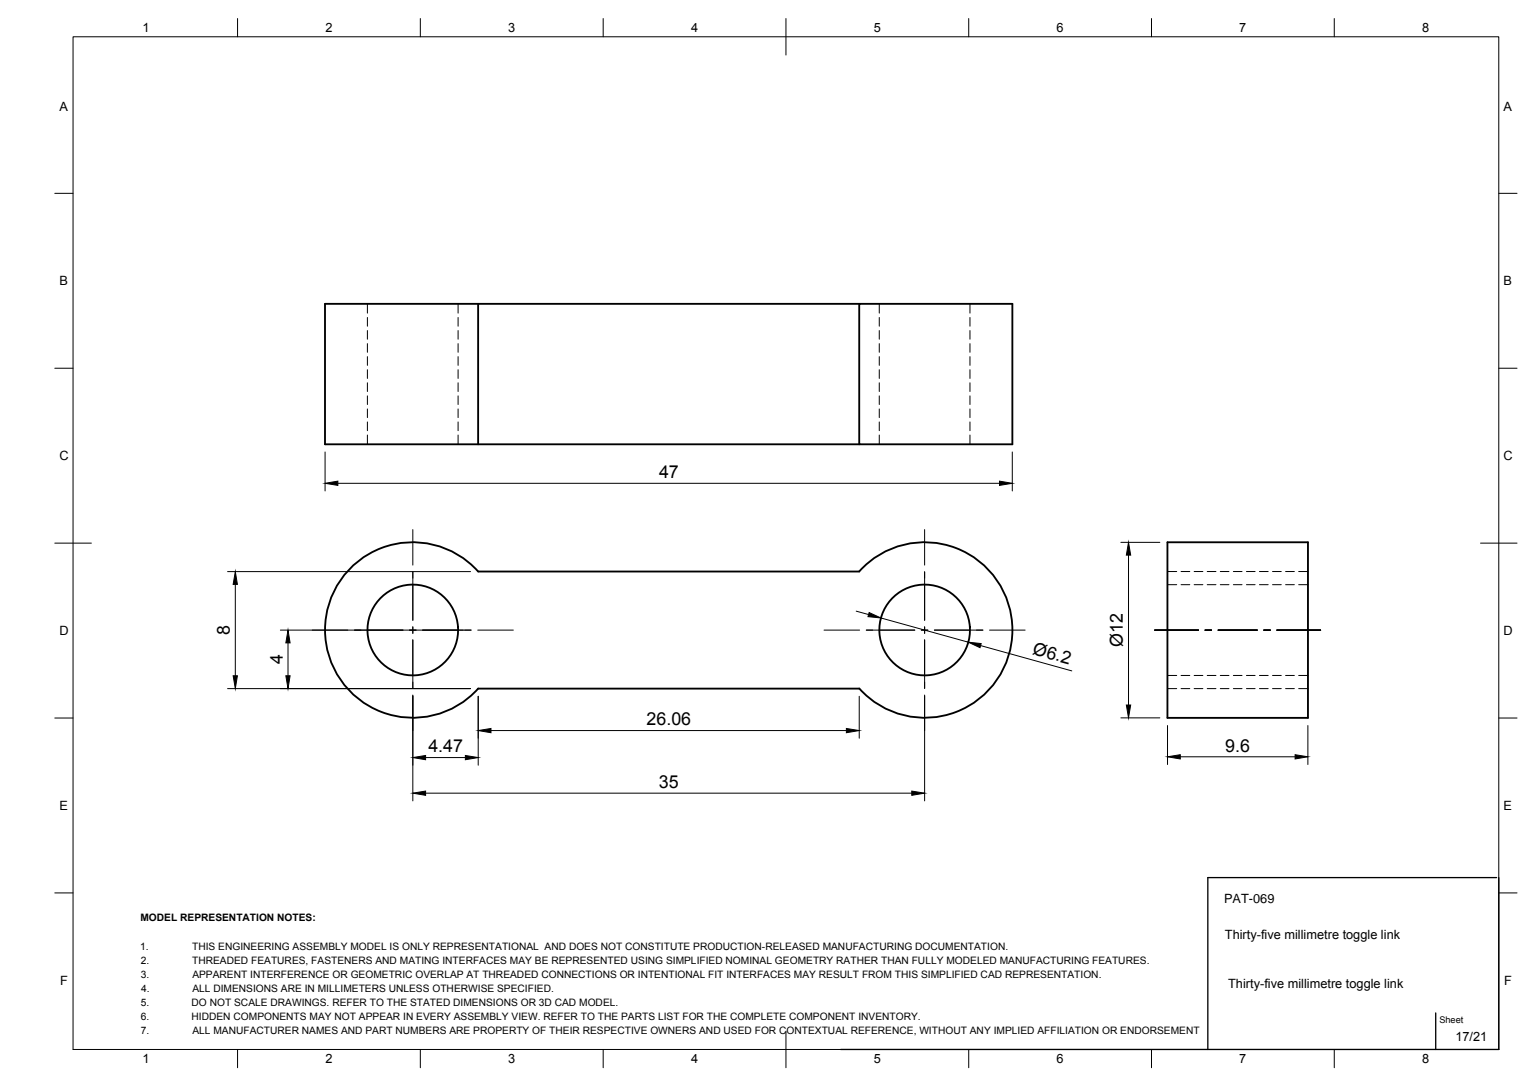
ISO-10303-21;
HEADER;
/* Generated by software containing ST-Developer
 * from STEP Tools, Inc. (www.steptools.com) 
 */

FILE_DESCRIPTION(
/* description */ ('Located fixture plate with toggle clamp'),
/* implementation_level */ '2;1');

FILE_NAME(
/* name */ 'Thirty-five millimetre toggle link.step',
/* time_stamp */ '2026-10-27T21:36:12-07:00',
/* author */ (''),
/* organization */ (''),
/* preprocessor_version */ 'ST-DEVELOPER v20.2',
/* originating_system */ 'Autodesk Translation Framework v15.17.0.0',
/* authorisation */ '');

FILE_SCHEMA (('AUTOMOTIVE_DESIGN { 1 0 10303 214 3 1 1 }'));
ENDSEC;

DATA;
#10=MECHANICAL_DESIGN_GEOMETRIC_PRESENTATION_REPRESENTATION('',(#336),#9285);
#288=SHAPE_REPRESENTATION_RELATIONSHIP('SRR','None',#9413,#312);
#312=ADVANCED_BREP_SHAPE_REPRESENTATION('',(#357),#9275);
#336=STYLED_ITEM('',(#9626),#357);
#357=MANIFOLD_SOLID_BREP('Body1',#5187);
#466=FACE_BOUND('',#1297,.T.);
#467=FACE_BOUND('',#1298,.T.);
#468=FACE_BOUND('',#1302,.T.);
#469=FACE_BOUND('',#1303,.T.);
#628=PLANE('',#5867);
#629=PLANE('',#5868);
#630=PLANE('',#5870);
#631=PLANE('',#5873);
#897=FACE_OUTER_BOUND('',#1292,.T.);
#898=FACE_OUTER_BOUND('',#1293,.T.);
#899=FACE_OUTER_BOUND('',#1294,.T.);
#900=FACE_OUTER_BOUND('',#1295,.T.);
#901=FACE_OUTER_BOUND('',#1296,.T.);
#902=FACE_OUTER_BOUND('',#1299,.T.);
#903=FACE_OUTER_BOUND('',#1300,.T.);
#904=FACE_OUTER_BOUND('',#1301,.T.);
#1292=EDGE_LOOP('',(#4498,#4499,#4500,#4501));
#1293=EDGE_LOOP('',(#4502,#4503,#4504,#4505));
#1294=EDGE_LOOP('',(#4506,#4507,#4508,#4509));
#1295=EDGE_LOOP('',(#4510,#4511,#4512,#4513));
#1296=EDGE_LOOP('',(#4514,#4515,#4516,#4517));
#1297=EDGE_LOOP('',(#4518));
#1298=EDGE_LOOP('',(#4519));
#1299=EDGE_LOOP('',(#4520,#4521,#4522,#4523));
#1300=EDGE_LOOP('',(#4524,#4525,#4526,#4527));
#1301=EDGE_LOOP('',(#4528,#4529,#4530,#4531));
#1302=EDGE_LOOP('',(#4532));
#1303=EDGE_LOOP('',(#4533));
#1536=CIRCLE('',#5859,0.31);
#1537=CIRCLE('',#5860,0.31);
#1538=CIRCLE('',#5862,0.31);
#1539=CIRCLE('',#5863,0.31);
#1540=CIRCLE('',#5865,0.6);
#1541=CIRCLE('',#5866,0.6);
#1542=CIRCLE('',#5869,0.6);
#1543=CIRCLE('',#5872,0.6);
#1913=LINE('',#8707,#2323);
#1914=LINE('',#8713,#2324);
#1915=LINE('',#8718,#2325);
#1916=LINE('',#8722,#2326);
#1917=LINE('',#8726,#2327);
#1918=LINE('',#8728,#2328);
#1919=LINE('',#8729,#2329);
#1920=LINE('',#8732,#2330);
#1921=LINE('',#8736,#2331);
#1922=LINE('',#8737,#2332);
#2323=VECTOR('',#7159,0.31);
#2324=VECTOR('',#7166,0.31);
#2325=VECTOR('',#7171,1.);
#2326=VECTOR('',#7174,1.);
#2327=VECTOR('',#7179,1.);
#2328=VECTOR('',#7180,1.);
#2329=VECTOR('',#7181,1.);
#2330=VECTOR('',#7184,1.);
#2331=VECTOR('',#7189,1.);
#2332=VECTOR('',#7190,1.);
#2734=VERTEX_POINT('',#8704);
#2735=VERTEX_POINT('',#8706);
#2736=VERTEX_POINT('',#8710);
#2737=VERTEX_POINT('',#8712);
#2738=VERTEX_POINT('',#8716);
#2739=VERTEX_POINT('',#8717);
#2740=VERTEX_POINT('',#8719);
#2741=VERTEX_POINT('',#8721);
#2742=VERTEX_POINT('',#8725);
#2743=VERTEX_POINT('',#8727);
#2744=VERTEX_POINT('',#8731);
#2745=VERTEX_POINT('',#8735);
#3337=EDGE_CURVE('',#2734,#2734,#1536,.T.);
#3338=EDGE_CURVE('',#2734,#2735,#1913,.T.);
#3339=EDGE_CURVE('',#2735,#2735,#1537,.T.);
#3340=EDGE_CURVE('',#2736,#2736,#1538,.T.);
#3341=EDGE_CURVE('',#2736,#2737,#1914,.T.);
#3342=EDGE_CURVE('',#2737,#2737,#1539,.T.);
#3343=EDGE_CURVE('',#2738,#2739,#1915,.T.);
#3344=EDGE_CURVE('',#2740,#2738,#1540,.T.);
#3345=EDGE_CURVE('',#2741,#2740,#1916,.T.);
#3346=EDGE_CURVE('',#2741,#2739,#1541,.T.);
#3347=EDGE_CURVE('',#2739,#2742,#1917,.T.);
#3348=EDGE_CURVE('',#2743,#2742,#1918,.T.);
#3349=EDGE_CURVE('',#2738,#2743,#1919,.T.);
#3350=EDGE_CURVE('',#2744,#2741,#1920,.T.);
#3351=EDGE_CURVE('',#2742,#2744,#1542,.T.);
#3352=EDGE_CURVE('',#2745,#2740,#1921,.T.);
#3353=EDGE_CURVE('',#2744,#2745,#1922,.T.);
#3354=EDGE_CURVE('',#2743,#2745,#1543,.T.);
#4498=ORIENTED_EDGE('',*,*,#3337,.F.);
#4499=ORIENTED_EDGE('',*,*,#3338,.T.);
#4500=ORIENTED_EDGE('',*,*,#3339,.F.);
#4501=ORIENTED_EDGE('',*,*,#3338,.F.);
#4502=ORIENTED_EDGE('',*,*,#3340,.F.);
#4503=ORIENTED_EDGE('',*,*,#3341,.T.);
#4504=ORIENTED_EDGE('',*,*,#3342,.F.);
#4505=ORIENTED_EDGE('',*,*,#3341,.F.);
#4506=ORIENTED_EDGE('',*,*,#3343,.F.);
#4507=ORIENTED_EDGE('',*,*,#3344,.F.);
#4508=ORIENTED_EDGE('',*,*,#3345,.F.);
#4509=ORIENTED_EDGE('',*,*,#3346,.T.);
#4510=ORIENTED_EDGE('',*,*,#3343,.T.);
#4511=ORIENTED_EDGE('',*,*,#3347,.T.);
#4512=ORIENTED_EDGE('',*,*,#3348,.F.);
#4513=ORIENTED_EDGE('',*,*,#3349,.F.);
#4514=ORIENTED_EDGE('',*,*,#3346,.F.);
#4515=ORIENTED_EDGE('',*,*,#3350,.F.);
#4516=ORIENTED_EDGE('',*,*,#3351,.F.);
#4517=ORIENTED_EDGE('',*,*,#3347,.F.);
#4518=ORIENTED_EDGE('',*,*,#3337,.T.);
#4519=ORIENTED_EDGE('',*,*,#3340,.T.);
#4520=ORIENTED_EDGE('',*,*,#3345,.T.);
#4521=ORIENTED_EDGE('',*,*,#3352,.F.);
#4522=ORIENTED_EDGE('',*,*,#3353,.F.);
#4523=ORIENTED_EDGE('',*,*,#3350,.T.);
#4524=ORIENTED_EDGE('',*,*,#3348,.T.);
#4525=ORIENTED_EDGE('',*,*,#3351,.T.);
#4526=ORIENTED_EDGE('',*,*,#3353,.T.);
#4527=ORIENTED_EDGE('',*,*,#3354,.F.);
#4528=ORIENTED_EDGE('',*,*,#3349,.T.);
#4529=ORIENTED_EDGE('',*,*,#3354,.T.);
#4530=ORIENTED_EDGE('',*,*,#3352,.T.);
#4531=ORIENTED_EDGE('',*,*,#3344,.T.);
#4532=ORIENTED_EDGE('',*,*,#3339,.T.);
#4533=ORIENTED_EDGE('',*,*,#3342,.T.);
#4855=CYLINDRICAL_SURFACE('',#5858,0.31);
#4856=CYLINDRICAL_SURFACE('',#5861,0.31);
#4857=CYLINDRICAL_SURFACE('',#5864,0.6);
#4858=CYLINDRICAL_SURFACE('',#5871,0.6);
#5098=ADVANCED_FACE('',(#897),#4855,.F.);
#5099=ADVANCED_FACE('',(#898),#4856,.F.);
#5100=ADVANCED_FACE('',(#899),#4857,.T.);
#5101=ADVANCED_FACE('',(#900),#628,.T.);
#5102=ADVANCED_FACE('',(#901,#466,#467),#629,.F.);
#5103=ADVANCED_FACE('',(#902),#630,.T.);
#5104=ADVANCED_FACE('',(#903),#4858,.T.);
#5105=ADVANCED_FACE('',(#904,#468,#469),#631,.T.);
#5187=CLOSED_SHELL('',(#5098,#5099,#5100,#5101,#5102,#5103,#5104,#5105));
#5857=AXIS2_PLACEMENT_3D('',#8702,#7153,#7154);
#5858=AXIS2_PLACEMENT_3D('',#8703,#7155,#7156);
#5859=AXIS2_PLACEMENT_3D('',#8705,#7157,#7158);
#5860=AXIS2_PLACEMENT_3D('',#8708,#7160,#7161);
#5861=AXIS2_PLACEMENT_3D('',#8709,#7162,#7163);
#5862=AXIS2_PLACEMENT_3D('',#8711,#7164,#7165);
#5863=AXIS2_PLACEMENT_3D('',#8714,#7167,#7168);
#5864=AXIS2_PLACEMENT_3D('',#8715,#7169,#7170);
#5865=AXIS2_PLACEMENT_3D('',#8720,#7172,#7173);
#5866=AXIS2_PLACEMENT_3D('',#8723,#7175,#7176);
#5867=AXIS2_PLACEMENT_3D('',#8724,#7177,#7178);
#5868=AXIS2_PLACEMENT_3D('',#8730,#7182,#7183);
#5869=AXIS2_PLACEMENT_3D('',#8733,#7185,#7186);
#5870=AXIS2_PLACEMENT_3D('',#8734,#7187,#7188);
#5871=AXIS2_PLACEMENT_3D('',#8738,#7191,#7192);
#5872=AXIS2_PLACEMENT_3D('',#8739,#7193,#7194);
#5873=AXIS2_PLACEMENT_3D('',#8740,#7195,#7196);
#7153=DIRECTION('axis',(0.,0.,1.));
#7154=DIRECTION('refdir',(1.,0.,0.));
#7155=DIRECTION('center_axis',(0.,1.,0.));
#7156=DIRECTION('ref_axis',(1.,0.,0.));
#7157=DIRECTION('center_axis',(0.,1.,0.));
#7158=DIRECTION('ref_axis',(1.,0.,0.));
#7159=DIRECTION('',(0.,1.,0.));
#7160=DIRECTION('center_axis',(0.,-1.,0.));
#7161=DIRECTION('ref_axis',(1.,0.,0.));
#7162=DIRECTION('center_axis',(0.,1.,0.));
#7163=DIRECTION('ref_axis',(1.,0.,0.));
#7164=DIRECTION('center_axis',(0.,1.,0.));
#7165=DIRECTION('ref_axis',(1.,0.,0.));
#7166=DIRECTION('',(0.,1.,0.));
#7167=DIRECTION('center_axis',(0.,-1.,0.));
#7168=DIRECTION('ref_axis',(1.,0.,0.));
#7169=DIRECTION('center_axis',(0.,1.,0.));
#7170=DIRECTION('ref_axis',(1.,0.,0.));
#7171=DIRECTION('',(0.,-1.,0.));
#7172=DIRECTION('center_axis',(0.,1.,0.));
#7173=DIRECTION('ref_axis',(1.,0.,0.));
#7174=DIRECTION('',(0.,1.,0.));
#7175=DIRECTION('center_axis',(0.,1.,0.));
#7176=DIRECTION('ref_axis',(1.,0.,0.));
#7177=DIRECTION('center_axis',(0.062254101962613,0.,-0.998060332238903));
#7178=DIRECTION('ref_axis',(-0.998060332238903,0.,-0.062254101962613));
#7179=DIRECTION('',(-0.998060332238903,0.,-0.062254101962613));
#7180=DIRECTION('',(0.,-1.,0.));
#7181=DIRECTION('',(-0.998060332238903,0.,-0.062254101962613));
#7182=DIRECTION('center_axis',(0.,1.,0.));
#7183=DIRECTION('ref_axis',(1.,0.,0.));
#7184=DIRECTION('',(0.998060332238903,0.,0.062254101962613));
#7185=DIRECTION('center_axis',(0.,1.,0.));
#7186=DIRECTION('ref_axis',(1.,0.,0.));
#7187=DIRECTION('center_axis',(-0.062254101962613,0.,0.998060332238903));
#7188=DIRECTION('ref_axis',(0.998060332238903,0.,0.062254101962613));
#7189=DIRECTION('',(0.998060332238903,0.,0.062254101962613));
#7190=DIRECTION('',(0.,1.,0.));
#7191=DIRECTION('center_axis',(0.,1.,0.));
#7192=DIRECTION('ref_axis',(-0.998060332238903,0.,-0.0622541019626133));
#7193=DIRECTION('center_axis',(0.,1.,0.));
#7194=DIRECTION('ref_axis',(1.,0.,0.));
#7195=DIRECTION('center_axis',(0.,1.,0.));
#7196=DIRECTION('ref_axis',(1.,0.,0.));
#8702=CARTESIAN_POINT('',(0.,0.,0.));
#8703=CARTESIAN_POINT('Origin',(2.49048674522936,-0.6,2.28211064313085));
#8704=CARTESIAN_POINT('',(2.18048674522936,-0.48,2.28211064313085));
#8705=CARTESIAN_POINT('Origin',(2.49048674522936,-0.48,2.28211064313085));
#8706=CARTESIAN_POINT('',(2.18048674522936,0.48,2.28211064313085));
#8707=CARTESIAN_POINT('',(2.18048674522936,-0.6,2.28211064313085));
#8708=CARTESIAN_POINT('Origin',(2.49048674522936,0.48,2.28211064313085));
#8709=CARTESIAN_POINT('Origin',(5.98369790806552,-0.6,2.5));
#8710=CARTESIAN_POINT('',(5.67369790806552,-0.48,2.5));
#8711=CARTESIAN_POINT('Origin',(5.98369790806552,-0.48,2.5));
#8712=CARTESIAN_POINT('',(5.67369790806552,0.48,2.5));
#8713=CARTESIAN_POINT('',(5.67369790806552,-0.6,2.5));
#8714=CARTESIAN_POINT('Origin',(5.98369790806552,0.48,2.5));
#8715=CARTESIAN_POINT('Origin',(5.98369790806552,-0.48,2.5));
#8716=CARTESIAN_POINT('',(5.56225339914413,0.48,2.07293498633112));
#8717=CARTESIAN_POINT('',(5.56225339914413,-0.48,2.07293498633112));
#8718=CARTESIAN_POINT('',(5.56225339914413,-0.48,2.07293498633112));
#8719=CARTESIAN_POINT('',(5.51245011757404,0.48,2.87138325212224));
#8720=CARTESIAN_POINT('Origin',(5.98369790806552,0.48,2.5));
#8721=CARTESIAN_POINT('',(5.51245011757404,-0.48,2.87138325212224));
#8722=CARTESIAN_POINT('',(5.51245011757404,-0.48,2.87138325212224));
#8723=CARTESIAN_POINT('Origin',(5.98369790806552,-0.48,2.5));
#8724=CARTESIAN_POINT('Origin',(6.00859954885057,-0.48,2.10077586710444));
#8725=CARTESIAN_POINT('',(2.96173453572085,-0.48,1.91072739100861));
#8726=CARTESIAN_POINT('',(6.00859954885057,-0.48,2.10077586710444));
#8727=CARTESIAN_POINT('',(2.96173453572085,0.48,1.91072739100861));
#8728=CARTESIAN_POINT('',(2.96173453572085,-0.48,1.91072739100861));
#8729=CARTESIAN_POINT('',(6.00859954885057,0.48,2.10077586710444));
#8730=CARTESIAN_POINT('Origin',(2.49048674522936,-0.48,2.28211064313085));
#8731=CARTESIAN_POINT('',(2.91193125415076,-0.48,2.70917565679974));
#8732=CARTESIAN_POINT('',(2.46558510444432,-0.48,2.68133477602642));
#8733=CARTESIAN_POINT('Origin',(2.49048674522936,-0.48,2.28211064313085));
#8734=CARTESIAN_POINT('Origin',(2.46558510444432,-0.48,2.68133477602642));
#8735=CARTESIAN_POINT('',(2.91193125415076,0.48,2.70917565679974));
#8736=CARTESIAN_POINT('',(2.46558510444432,0.48,2.68133477602642));
#8737=CARTESIAN_POINT('',(2.91193125415076,-0.48,2.70917565679974));
#8738=CARTESIAN_POINT('Origin',(2.49048674522936,-0.48,2.28211064313085));
#8739=CARTESIAN_POINT('Origin',(2.49048674522936,0.48,2.28211064313085));
#8740=CARTESIAN_POINT('Origin',(2.49048674522936,0.48,2.28211064313085));
#9245=UNCERTAINTY_MEASURE_WITH_UNIT(LENGTH_MEASURE(0.001),#9286,
'DISTANCE_ACCURACY_VALUE',
'Maximum model space distance between geometric entities at asserted c
onnectivities');
#9255=UNCERTAINTY_MEASURE_WITH_UNIT(LENGTH_MEASURE(0.001),#9286,
'DISTANCE_ACCURACY_VALUE',
'Maximum model space distance between geometric entities at asserted c
onnectivities');
#9275=(
GEOMETRIC_REPRESENTATION_CONTEXT(3)
GLOBAL_UNCERTAINTY_ASSIGNED_CONTEXT((#9245))
GLOBAL_UNIT_ASSIGNED_CONTEXT((#9286,#9288,#9289))
REPRESENTATION_CONTEXT('','3D')
);
#9285=(
GEOMETRIC_REPRESENTATION_CONTEXT(3)
GLOBAL_UNCERTAINTY_ASSIGNED_CONTEXT((#9255))
GLOBAL_UNIT_ASSIGNED_CONTEXT((#9286,#9288,#9289))
REPRESENTATION_CONTEXT('','3D')
);
#9286=(
LENGTH_UNIT()
NAMED_UNIT(*)
SI_UNIT(.CENTI.,.METRE.)
);
#9288=(
NAMED_UNIT(*)
PLANE_ANGLE_UNIT()
SI_UNIT($,.RADIAN.)
);
#9289=(
NAMED_UNIT(*)
SI_UNIT($,.STERADIAN.)
SOLID_ANGLE_UNIT()
);
#9309=SHAPE_DEFINITION_REPRESENTATION(#9338,#9413);
#9338=PRODUCT_DEFINITION_SHAPE('',$,#9443);
#9413=SHAPE_REPRESENTATION('',(#5857),#9275);
#9423=PRODUCT_DEFINITION_CONTEXT('part definition',#9512,'design');
#9443=PRODUCT_DEFINITION('Thirty-five millimetre toggle link',
'Thirty-five millimetre toggle link',#9472,#9423);
#9472=PRODUCT_DEFINITION_FORMATION('',$,#9533);
#9512=APPLICATION_CONTEXT(
'Core Data for Automotive Mechanical Design Process');
#9513=PRODUCT_CONTEXT('part definition',#9512,'mechanical');
#9533=PRODUCT('Thirty-five millimetre toggle link',
'Thirty-five millimetre toggle link',
'Thirty-five millimetre toggle link',(#9513));
#9620=COLOUR_RGB('Off White',0.89,0.88,0.83);
#9621=FILL_AREA_STYLE_COLOUR('',#9620);
#9622=FILL_AREA_STYLE('',(#9621));
#9623=SURFACE_STYLE_FILL_AREA(#9622);
#9624=SURFACE_SIDE_STYLE('',(#9623));
#9625=SURFACE_STYLE_USAGE(.BOTH.,#9624);
#9626=PRESENTATION_STYLE_ASSIGNMENT((#9625));
ENDSEC;
END-ISO-10303-21;
